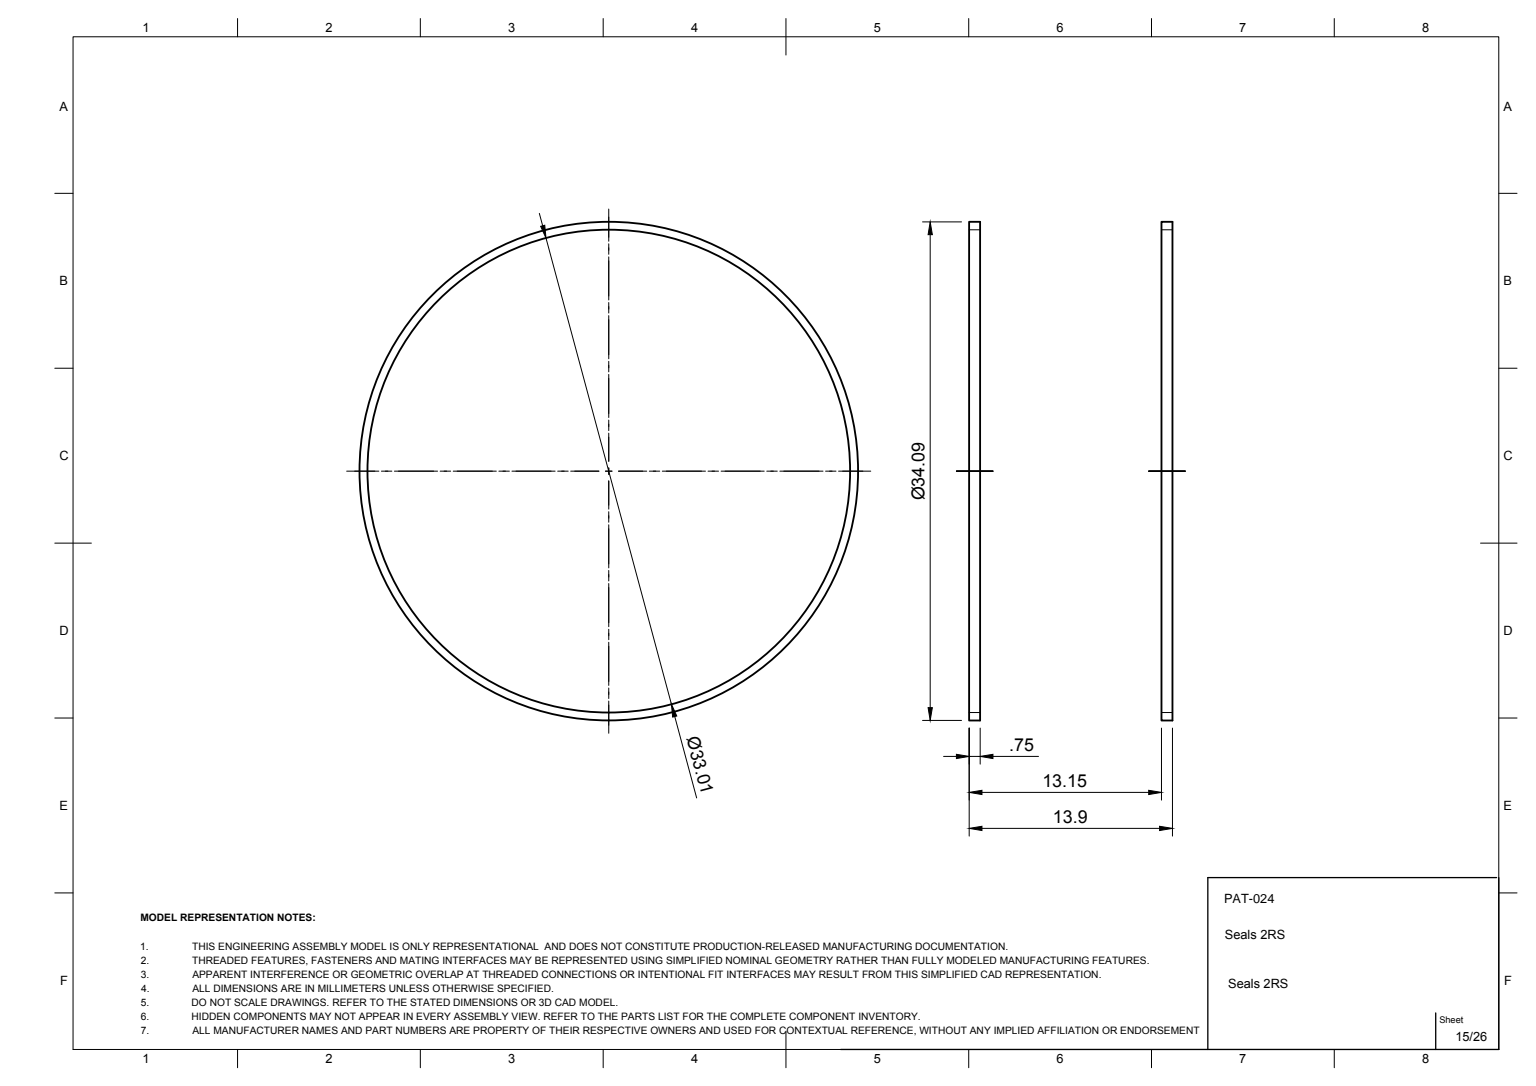
ISO-10303-21;
HEADER;
/* Generated by software containing ST-Developer
 * from STEP Tools, Inc. (www.steptools.com) 
 */

FILE_DESCRIPTION(
/* description */ ('Compact handwheel screw vise'),
/* implementation_level */ '2;1');

FILE_NAME(
/* name */ 'Seals 2RS.step',
/* time_stamp */ '2026-10-29T16:08:22-07:00',
/* author */ (''),
/* organization */ (''),
/* preprocessor_version */ 'ST-DEVELOPER v20.2',
/* originating_system */ 'Autodesk Translation Framework v15.17.0.0',
/* authorisation */ '');

FILE_SCHEMA (('AUTOMOTIVE_DESIGN { 1 0 10303 214 3 1 1 }'));
ENDSEC;

DATA;
#10=MECHANICAL_DESIGN_GEOMETRIC_PRESENTATION_REPRESENTATION('',(#662,#663),#25074);
#599=SHAPE_REPRESENTATION_RELATIONSHIP('SRR','None',#25208,#627);
#627=ADVANCED_BREP_SHAPE_REPRESENTATION('',(#697,#698),#25055);
#662=STYLED_ITEM('',(#25439),#697);
#663=STYLED_ITEM('',(#25439),#698);
#697=MANIFOLD_SOLID_BREP('Body1',#8071);
#698=MANIFOLD_SOLID_BREP('Body2',#8072);
#765=FACE_BOUND('',#1672,.T.);
#766=FACE_BOUND('',#1675,.T.);
#767=FACE_BOUND('',#1678,.T.);
#768=FACE_BOUND('',#1681,.T.);
#892=PLANE('',#8685);
#893=PLANE('',#8690);
#894=PLANE('',#8693);
#895=PLANE('',#8698);
#1148=FACE_OUTER_BOUND('',#1671,.T.);
#1149=FACE_OUTER_BOUND('',#1673,.T.);
#1150=FACE_OUTER_BOUND('',#1674,.T.);
#1151=FACE_OUTER_BOUND('',#1676,.T.);
#1152=FACE_OUTER_BOUND('',#1677,.T.);
#1153=FACE_OUTER_BOUND('',#1679,.T.);
#1154=FACE_OUTER_BOUND('',#1680,.T.);
#1155=FACE_OUTER_BOUND('',#1682,.T.);
#1671=EDGE_LOOP('',(#5719));
#1672=EDGE_LOOP('',(#5720));
#1673=EDGE_LOOP('',(#5721,#5722,#5723,#5724));
#1674=EDGE_LOOP('',(#5725));
#1675=EDGE_LOOP('',(#5726));
#1676=EDGE_LOOP('',(#5727,#5728,#5729,#5730));
#1677=EDGE_LOOP('',(#5731));
#1678=EDGE_LOOP('',(#5732));
#1679=EDGE_LOOP('',(#5733,#5734,#5735,#5736));
#1680=EDGE_LOOP('',(#5737));
#1681=EDGE_LOOP('',(#5738));
#1682=EDGE_LOOP('',(#5739,#5740,#5741,#5742));
#2191=LINE('',#12290,#2699);
#2192=LINE('',#12295,#2700);
#2193=LINE('',#12304,#2701);
#2194=LINE('',#12309,#2702);
#2699=VECTOR('',#9911,1.70469);
#2700=VECTOR('',#9918,1.65031);
#2701=VECTOR('',#9929,1.70469);
#2702=VECTOR('',#9936,1.65031);
#3211=CIRCLE('',#8686,1.70469);
#3212=CIRCLE('',#8687,1.65031);
#3213=CIRCLE('',#8689,1.70469);
#3214=CIRCLE('',#8691,1.65031);
#3215=CIRCLE('',#8694,1.70469);
#3216=CIRCLE('',#8695,1.65031);
#3217=CIRCLE('',#8697,1.70469);
#3218=CIRCLE('',#8699,1.65031);
#3528=VERTEX_POINT('',#12283);
#3529=VERTEX_POINT('',#12285);
#3530=VERTEX_POINT('',#12288);
#3531=VERTEX_POINT('',#12292);
#3532=VERTEX_POINT('',#12297);
#3533=VERTEX_POINT('',#12299);
#3534=VERTEX_POINT('',#12302);
#3535=VERTEX_POINT('',#12306);
#4346=EDGE_CURVE('',#3528,#3528,#3211,.T.);
#4347=EDGE_CURVE('',#3529,#3529,#3212,.T.);
#4348=EDGE_CURVE('',#3530,#3530,#3213,.T.);
#4349=EDGE_CURVE('',#3530,#3528,#2191,.T.);
#4350=EDGE_CURVE('',#3531,#3531,#3214,.T.);
#4351=EDGE_CURVE('',#3531,#3529,#2192,.T.);
#4352=EDGE_CURVE('',#3532,#3532,#3215,.T.);
#4353=EDGE_CURVE('',#3533,#3533,#3216,.T.);
#4354=EDGE_CURVE('',#3534,#3534,#3217,.T.);
#4355=EDGE_CURVE('',#3534,#3532,#2193,.T.);
#4356=EDGE_CURVE('',#3535,#3535,#3218,.T.);
#4357=EDGE_CURVE('',#3535,#3533,#2194,.T.);
#5719=ORIENTED_EDGE('',*,*,#4346,.F.);
#5720=ORIENTED_EDGE('',*,*,#4347,.T.);
#5721=ORIENTED_EDGE('',*,*,#4348,.F.);
#5722=ORIENTED_EDGE('',*,*,#4349,.T.);
#5723=ORIENTED_EDGE('',*,*,#4346,.T.);
#5724=ORIENTED_EDGE('',*,*,#4349,.F.);
#5725=ORIENTED_EDGE('',*,*,#4348,.T.);
#5726=ORIENTED_EDGE('',*,*,#4350,.F.);
#5727=ORIENTED_EDGE('',*,*,#4350,.T.);
#5728=ORIENTED_EDGE('',*,*,#4351,.T.);
#5729=ORIENTED_EDGE('',*,*,#4347,.F.);
#5730=ORIENTED_EDGE('',*,*,#4351,.F.);
#5731=ORIENTED_EDGE('',*,*,#4352,.F.);
#5732=ORIENTED_EDGE('',*,*,#4353,.T.);
#5733=ORIENTED_EDGE('',*,*,#4354,.F.);
#5734=ORIENTED_EDGE('',*,*,#4355,.T.);
#5735=ORIENTED_EDGE('',*,*,#4352,.T.);
#5736=ORIENTED_EDGE('',*,*,#4355,.F.);
#5737=ORIENTED_EDGE('',*,*,#4354,.T.);
#5738=ORIENTED_EDGE('',*,*,#4356,.F.);
#5739=ORIENTED_EDGE('',*,*,#4356,.T.);
#5740=ORIENTED_EDGE('',*,*,#4357,.T.);
#5741=ORIENTED_EDGE('',*,*,#4353,.F.);
#5742=ORIENTED_EDGE('',*,*,#4357,.F.);
#7386=CYLINDRICAL_SURFACE('',#8688,1.70469);
#7387=CYLINDRICAL_SURFACE('',#8692,1.65031);
#7388=CYLINDRICAL_SURFACE('',#8696,1.70469);
#7389=CYLINDRICAL_SURFACE('',#8700,1.65031);
#7718=ADVANCED_FACE('',(#1148,#765),#892,.T.);
#7719=ADVANCED_FACE('',(#1149),#7386,.T.);
#7720=ADVANCED_FACE('',(#1150,#766),#893,.T.);
#7721=ADVANCED_FACE('',(#1151),#7387,.F.);
#7722=ADVANCED_FACE('',(#1152,#767),#894,.T.);
#7723=ADVANCED_FACE('',(#1153),#7388,.T.);
#7724=ADVANCED_FACE('',(#1154,#768),#895,.T.);
#7725=ADVANCED_FACE('',(#1155),#7389,.F.);
#8071=CLOSED_SHELL('',(#7718,#7719,#7720,#7721));
#8072=CLOSED_SHELL('',(#7722,#7723,#7724,#7725));
#8684=AXIS2_PLACEMENT_3D('',#12281,#9899,#9900);
#8685=AXIS2_PLACEMENT_3D('',#12282,#9901,#9902);
#8686=AXIS2_PLACEMENT_3D('',#12284,#9903,#9904);
#8687=AXIS2_PLACEMENT_3D('',#12286,#9905,#9906);
#8688=AXIS2_PLACEMENT_3D('',#12287,#9907,#9908);
#8689=AXIS2_PLACEMENT_3D('',#12289,#9909,#9910);
#8690=AXIS2_PLACEMENT_3D('',#12291,#9912,#9913);
#8691=AXIS2_PLACEMENT_3D('',#12293,#9914,#9915);
#8692=AXIS2_PLACEMENT_3D('',#12294,#9916,#9917);
#8693=AXIS2_PLACEMENT_3D('',#12296,#9919,#9920);
#8694=AXIS2_PLACEMENT_3D('',#12298,#9921,#9922);
#8695=AXIS2_PLACEMENT_3D('',#12300,#9923,#9924);
#8696=AXIS2_PLACEMENT_3D('',#12301,#9925,#9926);
#8697=AXIS2_PLACEMENT_3D('',#12303,#9927,#9928);
#8698=AXIS2_PLACEMENT_3D('',#12305,#9930,#9931);
#8699=AXIS2_PLACEMENT_3D('',#12307,#9932,#9933);
#8700=AXIS2_PLACEMENT_3D('',#12308,#9934,#9935);
#9899=DIRECTION('axis',(0.,0.,1.));
#9900=DIRECTION('refdir',(1.,0.,0.));
#9901=DIRECTION('center_axis',(0.,1.,0.));
#9902=DIRECTION('ref_axis',(0.,0.,1.));
#9903=DIRECTION('center_axis',(0.,-1.,0.));
#9904=DIRECTION('ref_axis',(1.,0.,0.));
#9905=DIRECTION('center_axis',(0.,-1.,0.));
#9906=DIRECTION('ref_axis',(1.,0.,0.));
#9907=DIRECTION('center_axis',(0.,-1.,0.));
#9908=DIRECTION('ref_axis',(1.,0.,0.));
#9909=DIRECTION('center_axis',(0.,-1.,0.));
#9910=DIRECTION('ref_axis',(1.,0.,0.));
#9911=DIRECTION('',(0.,1.,0.));
#9912=DIRECTION('center_axis',(0.,-1.,0.));
#9913=DIRECTION('ref_axis',(0.,0.,-1.));
#9914=DIRECTION('center_axis',(0.,-1.,0.));
#9915=DIRECTION('ref_axis',(1.,0.,0.));
#9916=DIRECTION('center_axis',(0.,-1.,0.));
#9917=DIRECTION('ref_axis',(1.,0.,0.));
#9918=DIRECTION('',(0.,1.,0.));
#9919=DIRECTION('center_axis',(0.,1.,0.));
#9920=DIRECTION('ref_axis',(0.,0.,1.));
#9921=DIRECTION('center_axis',(0.,-1.,0.));
#9922=DIRECTION('ref_axis',(1.,0.,0.));
#9923=DIRECTION('center_axis',(0.,-1.,0.));
#9924=DIRECTION('ref_axis',(1.,0.,0.));
#9925=DIRECTION('center_axis',(0.,-1.,0.));
#9926=DIRECTION('ref_axis',(1.,0.,0.));
#9927=DIRECTION('center_axis',(0.,-1.,0.));
#9928=DIRECTION('ref_axis',(1.,0.,0.));
#9929=DIRECTION('',(0.,1.,0.));
#9930=DIRECTION('center_axis',(0.,-1.,0.));
#9931=DIRECTION('ref_axis',(0.,0.,-1.));
#9932=DIRECTION('center_axis',(0.,-1.,0.));
#9933=DIRECTION('ref_axis',(1.,0.,0.));
#9934=DIRECTION('center_axis',(0.,-1.,0.));
#9935=DIRECTION('ref_axis',(1.,0.,0.));
#9936=DIRECTION('',(0.,1.,0.));
#12281=CARTESIAN_POINT('',(0.,0.,0.));
#12282=CARTESIAN_POINT('Origin',(1.70469,0.695,0.));
#12283=CARTESIAN_POINT('',(-1.70469,0.695,-2.0876431520385E-16));
#12284=CARTESIAN_POINT('Origin',(0.,0.695,0.));
#12285=CARTESIAN_POINT('',(-1.65031,0.695,-2.02104685910087E-16));
#12286=CARTESIAN_POINT('Origin',(0.,0.695,0.));
#12287=CARTESIAN_POINT('Origin',(0.,0.6575,0.));
#12288=CARTESIAN_POINT('',(-1.70469,0.62,-2.0876431520385E-16));
#12289=CARTESIAN_POINT('Origin',(0.,0.62,0.));
#12290=CARTESIAN_POINT('',(-1.70469,0.6575,-2.0876431520385E-16));
#12291=CARTESIAN_POINT('Origin',(1.65031,0.62,0.));
#12292=CARTESIAN_POINT('',(-1.65031,0.62,-2.02104685910087E-16));
#12293=CARTESIAN_POINT('Origin',(0.,0.62,0.));
#12294=CARTESIAN_POINT('Origin',(0.,0.6575,0.));
#12295=CARTESIAN_POINT('',(-1.65031,0.6575,-2.02104685910087E-16));
#12296=CARTESIAN_POINT('Origin',(1.70469,-0.62,0.));
#12297=CARTESIAN_POINT('',(-1.70469,-0.62,-2.0876431520385E-16));
#12298=CARTESIAN_POINT('Origin',(0.,-0.62,0.));
#12299=CARTESIAN_POINT('',(-1.65031,-0.62,-2.02104685910087E-16));
#12300=CARTESIAN_POINT('Origin',(0.,-0.62,0.));
#12301=CARTESIAN_POINT('Origin',(0.,-0.6575,0.));
#12302=CARTESIAN_POINT('',(-1.70469,-0.695,-2.0876431520385E-16));
#12303=CARTESIAN_POINT('Origin',(0.,-0.695,0.));
#12304=CARTESIAN_POINT('',(-1.70469,-0.6575,-2.0876431520385E-16));
#12305=CARTESIAN_POINT('Origin',(1.65031,-0.695,0.));
#12306=CARTESIAN_POINT('',(-1.65031,-0.695,-2.02104685910087E-16));
#12307=CARTESIAN_POINT('Origin',(0.,-0.695,0.));
#12308=CARTESIAN_POINT('Origin',(0.,-0.6575,0.));
#12309=CARTESIAN_POINT('',(-1.65031,-0.6575,-2.02104685910087E-16));
#25021=UNCERTAINTY_MEASURE_WITH_UNIT(LENGTH_MEASURE(0.001),#25075,
'DISTANCE_ACCURACY_VALUE',
'Maximum model space distance between geometric entities at asserted c
onnectivities');
#25040=UNCERTAINTY_MEASURE_WITH_UNIT(LENGTH_MEASURE(0.001),#25075,
'DISTANCE_ACCURACY_VALUE',
'Maximum model space distance between geometric entities at asserted c
onnectivities');
#25055=(
GEOMETRIC_REPRESENTATION_CONTEXT(3)
GLOBAL_UNCERTAINTY_ASSIGNED_CONTEXT((#25021))
GLOBAL_UNIT_ASSIGNED_CONTEXT((#25075,#25077,#25078))
REPRESENTATION_CONTEXT('','3D')
);
#25074=(
GEOMETRIC_REPRESENTATION_CONTEXT(3)
GLOBAL_UNCERTAINTY_ASSIGNED_CONTEXT((#25040))
GLOBAL_UNIT_ASSIGNED_CONTEXT((#25075,#25077,#25078))
REPRESENTATION_CONTEXT('','3D')
);
#25075=(
LENGTH_UNIT()
NAMED_UNIT(*)
SI_UNIT(.CENTI.,.METRE.)
);
#25077=(
NAMED_UNIT(*)
PLANE_ANGLE_UNIT()
SI_UNIT($,.RADIAN.)
);
#25078=(
NAMED_UNIT(*)
SI_UNIT($,.STERADIAN.)
SOLID_ANGLE_UNIT()
);
#25093=SHAPE_DEFINITION_REPRESENTATION(#25126,#25208);
#25126=PRODUCT_DEFINITION_SHAPE('',$,#25242);
#25208=SHAPE_REPRESENTATION('',(#8684),#25055);
#25227=PRODUCT_DEFINITION_CONTEXT('part definition',#25328,'design');
#25242=PRODUCT_DEFINITION('Seals 2RS','Seals 2RS',#25275,#25227);
#25275=PRODUCT_DEFINITION_FORMATION('',$,#25344);
#25328=APPLICATION_CONTEXT(
'Core Data for Automotive Mechanical Design Process');
#25329=PRODUCT_CONTEXT('part definition',#25328,'mechanical');
#25344=PRODUCT('Seals 2RS','Seals 2RS','Seals 2RS',(#25329));
#25433=COLOUR_RGB('Grey',0.48,0.52,0.57);
#25434=FILL_AREA_STYLE_COLOUR('',#25433);
#25435=FILL_AREA_STYLE('',(#25434));
#25436=SURFACE_STYLE_FILL_AREA(#25435);
#25437=SURFACE_SIDE_STYLE('',(#25436));
#25438=SURFACE_STYLE_USAGE(.BOTH.,#25437);
#25439=PRESENTATION_STYLE_ASSIGNMENT((#25438));
ENDSEC;
END-ISO-10303-21;
